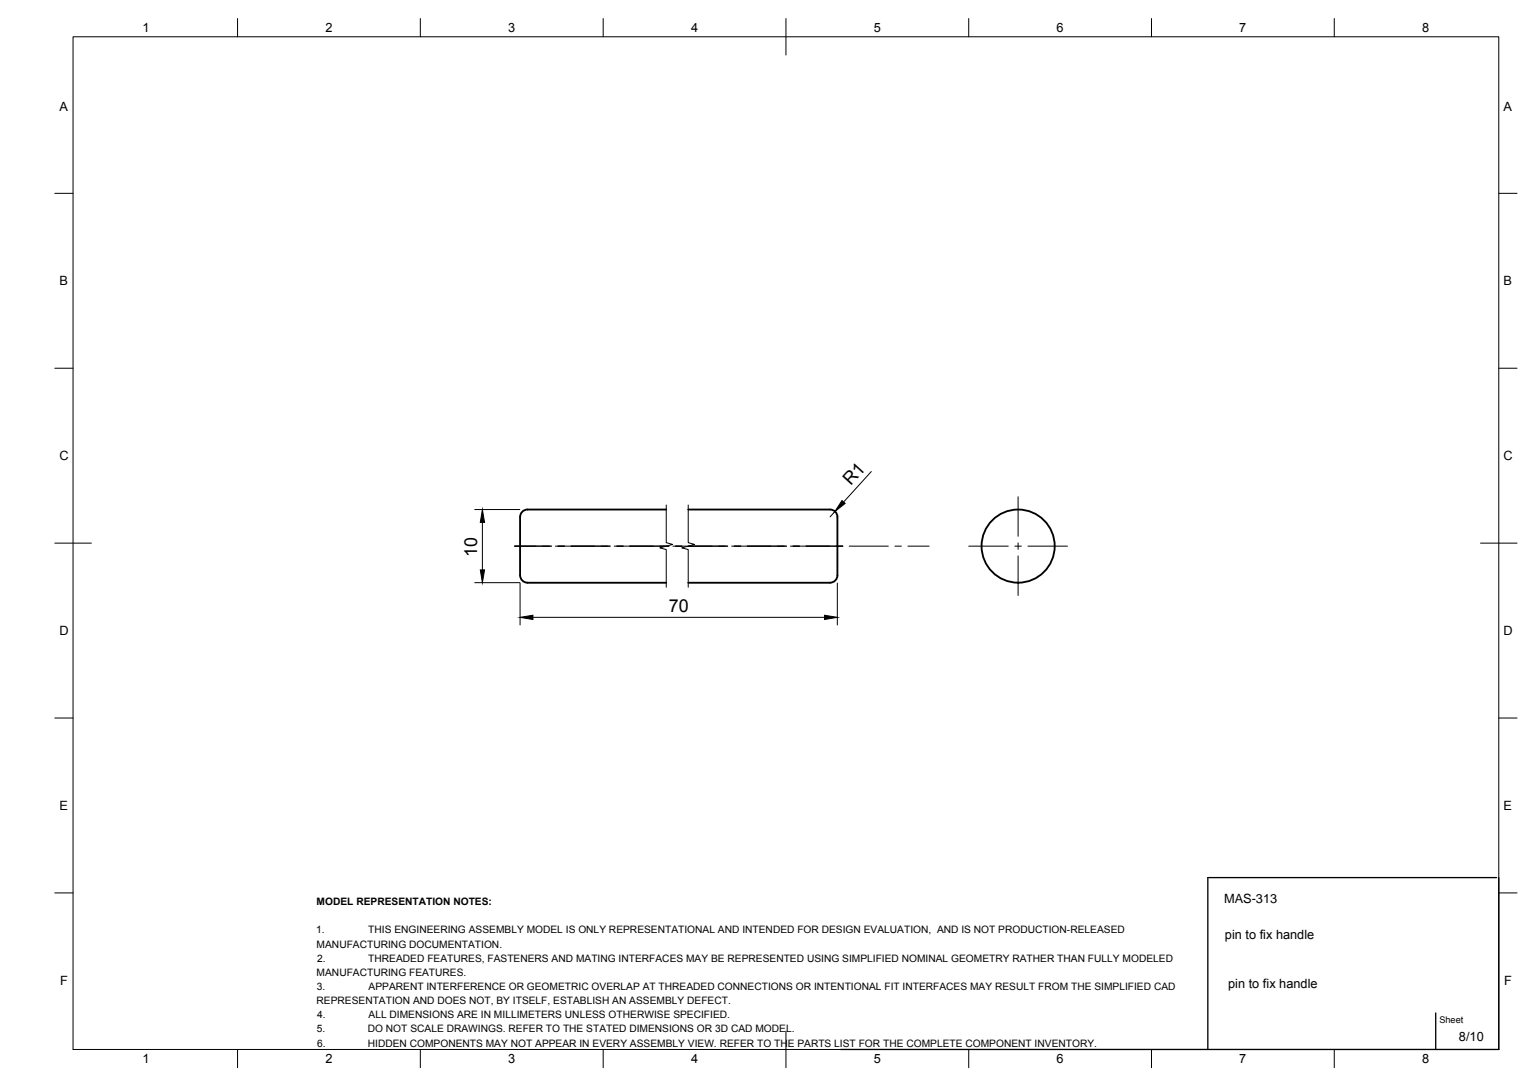
ISO-10303-21;
HEADER;
FILE_DESCRIPTION (('STEP AP214'),
    '1' );
FILE_NAME ('pin to fix handle.step',
    '2026-10-06T09:36:00',
    ( '' ),
    ( '' ),
    'SwSTEP 2.0',
    'SolidWorks 2025',
    '' );
FILE_SCHEMA (( 'AUTOMOTIVE_DESIGN' ));
ENDSEC;

DATA;
#87=VECTOR ( 'NONE', #10625, 1000.000000000000000 ) ;
#136=AXIS2_PLACEMENT_3D ( 'NONE', #2557, #579, #5269 ) ;
#167=DIRECTION ( 'NONE',  ( 1.000000000000000000, -1.876626137810916309E-30, 2.081668171172161734E-17 ) ) ;
#230=( LENGTH_UNIT ( ) NAMED_UNIT ( * ) SI_UNIT ( .MILLI., .METRE. ) );
#266=VECTOR ( 'NONE', #3751, 1000.000000000000000 ) ;
#291=PLANE ( 'NONE',  #9364 ) ;
#310=CARTESIAN_POINT ( 'NONE',  ( -823.8285638327238303, 78.67432280806536937, -89.68077099980398259 ) ) ;
#349=EDGE_CURVE ( 'NONE', #7831, #3787, #3152, .T. ) ;
#417=DIRECTION ( 'NONE',  ( 2.081668171172161734E-17, 4.930380657631307143E-31, -1.000000000000000000 ) ) ;
#440=CIRCLE ( 'NONE', #6189, 4.000000000000003553 ) ;
#493=EDGE_LOOP ( 'NONE', ( #7203, #9839, #8059, #6199 ) ) ;
#515=ORIENTED_EDGE ( 'NONE', *, *, #1701, .T. ) ;
#579=DIRECTION ( 'NONE',  ( -2.081668171172161734E-17, -4.930380657631307143E-31, 1.000000000000000000 ) ) ;
#638=CIRCLE ( 'NONE', #2031, 1.000000000000000888 ) ;
#710=DIRECTION ( 'NONE',  ( 1.000000000000000000, 0.000000000000000000, 0.000000000000000000 ) ) ;
#807=EDGE_CURVE ( 'NONE', #7831, #11221, #10092, .T. ) ;
#835=AXIS2_PLACEMENT_3D ( 'NONE', #1633, #2618, #6521 ) ;
#869=DIRECTION ( 'NONE',  ( 1.000000000000000000, -1.876626137810916309E-30, 2.081668171172161734E-17 ) ) ;
#886=ORIENTED_EDGE ( 'NONE', *, *, #1701, .F. ) ;
#924=LINE ( 'NONE', #5726, #266 ) ;
#977=DIRECTION ( 'NONE',  ( 1.000000000000000000, 0.000000000000000000, 0.000000000000000000 ) ) ;
#1010=CARTESIAN_POINT ( 'NONE',  ( -827.8285638327242850, 78.67432280806536937, -90.68077099980378364 ) ) ;
#1092=ORIENTED_EDGE ( 'NONE', *, *, #349, .F. ) ;
#1112=CARTESIAN_POINT ( 'NONE',  ( -818.8285638327247398, 78.67432280806536937, -158.6807709998041673 ) ) ;
#1184=SHAPE_REPRESENTATION_RELATIONSHIP ( 'NONE' , 'NONE' ,  #4872, #6043 ) ;
#1237=PRESENTATION_STYLE_ASSIGNMENT (( #7913 ) ) ;
#1300=DIRECTION ( 'NONE',  ( 1.000000000000000000, 0.000000000000000000, 0.000000000000000000 ) ) ;
#1388=ADVANCED_FACE ( 'NONE', ( #3889 ), #291, .F. ) ;
#1476=AXIS2_PLACEMENT_3D ( 'NONE', #10075, #7237, #11202 ) ;
#1505=ORIENTED_EDGE ( 'NONE', *, *, #349, .T. ) ;
#1609=CIRCLE ( 'NONE', #4593, 1.000000000000000888 ) ;
#1633=CARTESIAN_POINT ( 'NONE',  ( -823.8285638327242850, 78.67432280806536937, -90.68077099980378364 ) ) ;
#1659=CIRCLE ( 'NONE', #8766, 1.000000000000000888 ) ;
#1663=EDGE_LOOP ( 'NONE', ( #9512, #6396, #1868, #515 ) ) ;
#1669=CARTESIAN_POINT ( 'NONE',  ( -823.8285638327247398, 78.67432280806536937, -158.6807709998041673 ) ) ;
#1701=EDGE_CURVE ( 'NONE', #6923, #10076, #8157, .T. ) ;
#1727=ORIENTED_EDGE ( 'NONE', *, *, #11837, .F. ) ;
#1868=ORIENTED_EDGE ( 'NONE', *, *, #2750, .T. ) ;
#1872=PRODUCT_DEFINITION ( 'UNKNOWN', '', #5446, #1966 ) ;
#1966=PRODUCT_DEFINITION_CONTEXT ( 'detailed design', #7796, 'design' ) ;
#1972=AXIS2_PLACEMENT_3D ( 'NONE', #1669, #2530, #11129 ) ;
#2031=AXIS2_PLACEMENT_3D ( 'NONE', #6574, #2608, #7434 ) ;
#2069=EDGE_CURVE ( 'NONE', #10717, #3207, #440, .T. ) ;
#2234=CYLINDRICAL_SURFACE ( 'NONE', #9598, 5.000000000000115463 ) ;
#2273=CIRCLE ( 'NONE', #11162, 4.000000000000003553 ) ;
#2346=CARTESIAN_POINT ( 'NONE',  ( -823.8285638327245124, 78.67432280806536937, -159.6807709998044800 ) ) ;
#2363=( GEOMETRIC_REPRESENTATION_CONTEXT ( 3 ) GLOBAL_UNCERTAINTY_ASSIGNED_CONTEXT ( ( #10663 ) ) GLOBAL_UNIT_ASSIGNED_CONTEXT ( ( #230, #3198, #4081 ) ) REPRESENTATION_CONTEXT ( 'NONE', 'WORKASPACE' ) );
#2380=CARTESIAN_POINT ( 'NONE',  ( -818.8285638327237166, 78.67432280806536937, -89.68077099980398259 ) ) ;
#2394=FILL_AREA_STYLE ('',( #5928 ) ) ;
#2489=EDGE_LOOP ( 'NONE', ( #2863, #8978, #5125, #1092 ) ) ;
#2530=DIRECTION ( 'NONE',  ( -2.081668171172161734E-17, -4.930380657631307143E-31, 1.000000000000000000 ) ) ;
#2557=CARTESIAN_POINT ( 'NONE',  ( -823.8285638327247398, 78.67432280806536937, -158.6807709998041673 ) ) ;
#2608=DIRECTION ( 'NONE',  ( 1.224646799147376133E-16, 1.000000000000000000, 4.955873740258437191E-31 ) ) ;
#2618=DIRECTION ( 'NONE',  ( 2.081668171172161734E-17, 4.930380657631307143E-31, -1.000000000000000000 ) ) ;
#2750=EDGE_CURVE ( 'NONE', #11221, #6923, #924, .T. ) ;
#2778=DIRECTION ( 'NONE',  ( -2.081668171172161734E-17, -4.930380657631308019E-31, 1.000000000000000000 ) ) ;
#2790=CARTESIAN_POINT ( 'NONE',  ( -827.8285638327238303, 78.67432280806536937, -89.68077099980398259 ) ) ;
#2863=ORIENTED_EDGE ( 'NONE', *, *, #10666, .F. ) ;
#2903=EDGE_CURVE ( 'NONE', #11221, #8948, #1659, .T. ) ;
#3006=DIRECTION ( 'NONE',  ( 1.000000000000000000, -1.026341648675396322E-47, 2.081668171172161734E-17 ) ) ;
#3015=DIRECTION ( 'NONE',  ( 1.000000000000000000, 0.000000000000000000, 0.000000000000000000 ) ) ;
#3104=TOROIDAL_SURFACE ( 'NONE', #136, 4.000000000000045297, 1.000000000000000000 ) ;
#3152=CIRCLE ( 'NONE', #11256, 1.000000000000000888 ) ;
#3198=( NAMED_UNIT ( * ) PLANE_ANGLE_UNIT ( ) SI_UNIT ( $, .RADIAN. ) );
#3207=VERTEX_POINT ( 'NONE', #5427 ) ;
#3215=CARTESIAN_POINT ( 'NONE',  ( -823.8285638327242850, 78.67432280806536937, -90.68077099980378364 ) ) ;
#3400=ORIENTED_EDGE ( 'NONE', *, *, #2069, .T. ) ;
#3449=AXIS2_PLACEMENT_3D ( 'NONE', #7914, #9817, #5175 ) ;
#3543=DIRECTION ( 'NONE',  ( -2.081668171172161734E-17, -4.930380657631307143E-31, 1.000000000000000000 ) ) ;
#3642=FACE_OUTER_BOUND ( 'NONE', #1663, .T. ) ;
#3643=EDGE_LOOP ( 'NONE', ( #11417, #7051, #4704, #5616 ) ) ;
#3745=CARTESIAN_POINT ( 'NONE',  ( -823.8285638327247398, 78.67432280806536937, -158.6807709998041673 ) ) ;
#3751=DIRECTION ( 'NONE',  ( 2.081668171172161734E-17, 4.930380657631307143E-31, -1.000000000000000000 ) ) ;
#3787=VERTEX_POINT ( 'NONE', #7173 ) ;
#3807=ADVANCED_FACE ( 'NONE', ( #10268 ), #10840, .T. ) ;
#3889=FACE_OUTER_BOUND ( 'NONE', #4143, .T. ) ;
#3982=MANIFOLD_SOLID_BREP ( 'Fillet6', #4544 ) ;
#4081=( NAMED_UNIT ( * ) SI_UNIT ( $, .STERADIAN. ) SOLID_ANGLE_UNIT ( ) );
#4143=EDGE_LOOP ( 'NONE', ( #10187, #3400 ) ) ;
#4253=CARTESIAN_POINT ( 'NONE',  ( -823.8285638327238303, 78.67432280806536937, -89.68077099980398259 ) ) ;
#4432=DIRECTION ( 'NONE',  ( 1.000000000000000000, 0.000000000000000000, 0.000000000000000000 ) ) ;
#4501=AXIS2_PLACEMENT_3D ( 'NONE', #3215, #4892, #5819 ) ;
#4518=AXIS2_PLACEMENT_3D ( 'NONE', #11410, #6710, #3006 ) ;
#4544=CLOSED_SHELL ( 'NONE', ( #4609, #3807, #12155, #11684, #8450, #1388, #10453, #8041 ) ) ;
#4593=AXIS2_PLACEMENT_3D ( 'NONE', #10809, #8718, #7039 ) ;
#4609=ADVANCED_FACE ( 'NONE', ( #7576 ), #9837, .T. ) ;
#4626=CARTESIAN_POINT ( 'NONE',  ( -823.8285638327247398, 78.67432280806536937, -158.6807709998041673 ) ) ;
#4687=DIRECTION ( 'NONE',  ( 1.000000000000000000, 0.000000000000000000, 0.000000000000000000 ) ) ;
#4693=UNCERTAINTY_MEASURE_WITH_UNIT (LENGTH_MEASURE( 1.000000000000000082E-05 ), #8076, 'distance_accuracy_value', 'NONE');
#4699=CIRCLE ( 'NONE', #9621, 5.000000000000115463 ) ;
#4704=ORIENTED_EDGE ( 'NONE', *, *, #10020, .T. ) ;
#4754=FACE_OUTER_BOUND ( 'NONE', #8581, .T. ) ;
#4872=SHAPE_REPRESENTATION ( 'pin to fix handle', ( #11957 ), #10774 ) ;
#4885=EDGE_CURVE ( 'NONE', #3207, #10076, #1609, .T. ) ;
#4892=DIRECTION ( 'NONE',  ( -2.081668171172161734E-17, -4.930380657631307143E-31, 1.000000000000000000 ) ) ;
#5007=FACE_OUTER_BOUND ( 'NONE', #3643, .T. ) ;
#5035=AXIS2_PLACEMENT_3D ( 'NONE', #2346, #10626, #1300 ) ;
#5051=SURFACE_STYLE_FILL_AREA ( #2394 ) ;
#5118=STYLED_ITEM ( 'NONE', ( #1237 ), #3982 ) ;
#5125=ORIENTED_EDGE ( 'NONE', *, *, #11852, .F. ) ;
#5157=ORIENTED_EDGE ( 'NONE', *, *, #807, .F. ) ;
#5175=DIRECTION ( 'NONE',  ( 1.000000000000000000, 0.000000000000000000, 0.000000000000000000 ) ) ;
#5269=DIRECTION ( 'NONE',  ( 1.000000000000000000, -1.026341648675396322E-47, 2.081668171172161734E-17 ) ) ;
#5427=CARTESIAN_POINT ( 'NONE',  ( -819.8285638327245124, 78.67432280806536937, -159.6807709998044800 ) ) ;
#5446=PRODUCT_DEFINITION_FORMATION_WITH_SPECIFIED_SOURCE ( 'ANY', '', #7932, .NOT_KNOWN. ) ;
#5583=CARTESIAN_POINT ( 'NONE',  ( -818.8285638327242850, 78.67432280806536937, -90.68077099980378364 ) ) ;
#5590=DIRECTION ( 'NONE',  ( 2.081668171172161734E-17, 4.930380657631307143E-31, -1.000000000000000000 ) ) ;
#5616=ORIENTED_EDGE ( 'NONE', *, *, #2750, .F. ) ;
#5726=CARTESIAN_POINT ( 'NONE',  ( -828.8285638327239440, 78.67432280806536937, -89.68077099980398259 ) ) ;
#5735=PLANE ( 'NONE',  #7666 ) ;
#5784=ORIENTED_EDGE ( 'NONE', *, *, #11852, .T. ) ;
#5819=DIRECTION ( 'NONE',  ( 1.000000000000000000, -1.026341648675396322E-47, 2.081668171172161734E-17 ) ) ;
#5857=DIRECTION ( 'NONE',  ( -2.081668171172161734E-17, -4.930380657631308019E-31, 1.000000000000000000 ) ) ;
#5864=( NAMED_UNIT ( * ) PLANE_ANGLE_UNIT ( ) SI_UNIT ( $, .RADIAN. ) );
#5928=FILL_AREA_STYLE_COLOUR ( '', #9661 ) ;
#5979=EDGE_CURVE ( 'NONE', #10717, #6923, #638, .T. ) ;
#6032=CIRCLE ( 'NONE', #5035, 4.000000000000003553 ) ;
#6043=ADVANCED_BREP_SHAPE_REPRESENTATION ( '', ( #3982, #11957 ), #10774 ) ;
#6111=MECHANICAL_DESIGN_GEOMETRIC_PRESENTATION_REPRESENTATION('',(#5118),#2363);
#6132=APPLICATION_CONTEXT ( 'automotive_design' ) ;
#6189=AXIS2_PLACEMENT_3D ( 'NONE', #7587, #11482, #3015 ) ;
#6199=ORIENTED_EDGE ( 'NONE', *, *, #4885, .F. ) ;
#6267=CARTESIAN_POINT ( 'NONE',  ( -828.8285638327242850, 78.67432280806536937, -90.68077099980378364 ) ) ;
#6396=ORIENTED_EDGE ( 'NONE', *, *, #807, .T. ) ;
#6521=DIRECTION ( 'NONE',  ( 1.000000000000000000, 0.000000000000000000, 0.000000000000000000 ) ) ;
#6569=DIRECTION ( 'NONE',  ( 1.224646799147376133E-16, 1.000000000000000000, 4.955873740258437191E-31 ) ) ;
#6574=CARTESIAN_POINT ( 'NONE',  ( -827.8285638327247398, 78.67432280806536937, -158.6807709998041673 ) ) ;
#6624=ORIENTED_EDGE ( 'NONE', *, *, #2903, .F. ) ;
#6710=DIRECTION ( 'NONE',  ( -2.081668171172161734E-17, -4.930380657631307143E-31, 1.000000000000000000 ) ) ;
#6808=DIRECTION ( 'NONE',  ( -1.000000000000000000, 0.000000000000000000, 0.000000000000000000 ) ) ;
#6838=CARTESIAN_POINT ( 'NONE',  ( -819.8285638327242850, 78.67432280806536937, -90.68077099980378364 ) ) ;
#6866=TOROIDAL_SURFACE ( 'NONE', #4501, 4.000000000000045297, 1.000000000000000000 ) ;
#6889=EDGE_CURVE ( 'NONE', #7831, #10076, #11496, .T. ) ;
#6923=VERTEX_POINT ( 'NONE', #9178 ) ;
#7039=DIRECTION ( 'NONE',  ( 1.000000000000000000, 0.000000000000000000, 0.000000000000000000 ) ) ;
#7051=ORIENTED_EDGE ( 'NONE', *, *, #6889, .T. ) ;
#7173=CARTESIAN_POINT ( 'NONE',  ( -819.8285638327238303, 78.67432280806536937, -89.68077099980398259 ) ) ;
#7203=ORIENTED_EDGE ( 'NONE', *, *, #2069, .F. ) ;
#7237=DIRECTION ( 'NONE',  ( 2.081668171172161734E-17, 4.930380657631307143E-31, -1.000000000000000000 ) ) ;
#7380=EDGE_LOOP ( 'NONE', ( #8495, #1727, #7424, #886 ) ) ;
#7397=DIRECTION ( 'NONE',  ( -2.081668171172161734E-17, -4.930380657631307143E-31, 1.000000000000000000 ) ) ;
#7423=CYLINDRICAL_SURFACE ( 'NONE', #1476, 5.000000000000115463 ) ;
#7424=ORIENTED_EDGE ( 'NONE', *, *, #4885, .T. ) ;
#7434=DIRECTION ( 'NONE',  ( -1.000000000000000000, 0.000000000000000000, 0.000000000000000000 ) ) ;
#7439=DIRECTION ( 'NONE',  ( 1.000000000000000000, 0.000000000000000000, 0.000000000000000000 ) ) ;
#7576=FACE_OUTER_BOUND ( 'NONE', #2489, .T. ) ;
#7587=CARTESIAN_POINT ( 'NONE',  ( -823.8285638327245124, 78.67432280806536937, -159.6807709998044800 ) ) ;
#7637=SHAPE_DEFINITION_REPRESENTATION ( #8521, #4872 ) ;
#7658=EDGE_CURVE ( 'NONE', #8948, #3787, #2273, .T. ) ;
#7666=AXIS2_PLACEMENT_3D ( 'NONE', #11300, #2778, #869 ) ;
#7796=APPLICATION_CONTEXT ( 'automotive_design' ) ;
#7831=VERTEX_POINT ( 'NONE', #5583 ) ;
#7913=SURFACE_STYLE_USAGE ( .BOTH. , #10743 ) ;
#7914=CARTESIAN_POINT ( 'NONE',  ( -823.8285638327238303, 78.67432280806536937, -89.68077099980398259 ) ) ;
#7932=PRODUCT ( 'pin to fix handle', 'pin to fix handle', '', ( #11342 ) ) ;
#7955=DIRECTION ( 'NONE',  ( 1.000000000000000000, 0.000000000000000000, 0.000000000000000000 ) ) ;
#8041=ADVANCED_FACE ( 'NONE', ( #10822 ), #6866, .T. ) ;
#8059=ORIENTED_EDGE ( 'NONE', *, *, #10020, .F. ) ;
#8076=( LENGTH_UNIT ( ) NAMED_UNIT ( * ) SI_UNIT ( .MILLI., .METRE. ) );
#8157=CIRCLE ( 'NONE', #9541, 5.000000000000115463 ) ;
#8196=CARTESIAN_POINT ( 'NONE',  ( -827.8285638327245124, 78.67432280806536937, -159.6807709998044800 ) ) ;
#8323=FACE_OUTER_BOUND ( 'NONE', #7380, .T. ) ;
#8450=ADVANCED_FACE ( 'NONE', ( #4754 ), #5735, .T. ) ;
#8495=ORIENTED_EDGE ( 'NONE', *, *, #5979, .F. ) ;
#8498=DIRECTION ( 'NONE',  ( -1.000000000000000000, 0.000000000000000000, 0.000000000000000000 ) ) ;
#8521=PRODUCT_DEFINITION_SHAPE ( 'NONE', 'NONE',  #1872 ) ;
#8581=EDGE_LOOP ( 'NONE', ( #5784, #11546 ) ) ;
#8718=DIRECTION ( 'NONE',  ( -1.876626137810916309E-30, -1.000000000000000000, -4.930380657631307143E-31 ) ) ;
#8766=AXIS2_PLACEMENT_3D ( 'NONE', #1010, #6569, #8498 ) ;
#8948=VERTEX_POINT ( 'NONE', #2790 ) ;
#8978=ORIENTED_EDGE ( 'NONE', *, *, #2903, .T. ) ;
#9048=CARTESIAN_POINT ( 'NONE',  ( 0.000000000000000000, 0.000000000000000000, 0.000000000000000000 ) ) ;
#9105=CARTESIAN_POINT ( 'NONE',  ( -823.8285638327242850, 78.67432280806536937, -90.68077099980378364 ) ) ;
#9178=CARTESIAN_POINT ( 'NONE',  ( -828.8285638327247398, 78.67432280806536937, -158.6807709998041673 ) ) ;
#9364=AXIS2_PLACEMENT_3D ( 'NONE', #9577, #5857, #167 ) ;
#9440=DIRECTION ( 'NONE',  ( -1.876626137810916309E-30, -1.000000000000000000, -4.930380657631307143E-31 ) ) ;
#9512=ORIENTED_EDGE ( 'NONE', *, *, #6889, .F. ) ;
#9541=AXIS2_PLACEMENT_3D ( 'NONE', #4626, #3543, #4432 ) ;
#9577=CARTESIAN_POINT ( 'NONE',  ( -823.8285638327245124, 78.67432280806536937, -159.6807709998044800 ) ) ;
#9598=AXIS2_PLACEMENT_3D ( 'NONE', #310, #417, #6808 ) ;
#9621=AXIS2_PLACEMENT_3D ( 'NONE', #9105, #5590, #710 ) ;
#9661=COLOUR_RGB ( '', 0.72549020, 0.75294118, 0.79215686) ;
#9817=DIRECTION ( 'NONE',  ( -2.081668171172161734E-17, -4.930380657631307143E-31, 1.000000000000000000 ) ) ;
#9837=TOROIDAL_SURFACE ( 'NONE', #4518, 4.000000000000045297, 1.000000000000000000 ) ;
#9839=ORIENTED_EDGE ( 'NONE', *, *, #5979, .T. ) ;
#9973=CIRCLE ( 'NONE', #3449, 4.000000000000003553 ) ;
#10001=EDGE_LOOP ( 'NONE', ( #6624, #5157, #1505, #11857 ) ) ;
#10020=EDGE_CURVE ( 'NONE', #10076, #6923, #11591, .T. ) ;
#10075=CARTESIAN_POINT ( 'NONE',  ( -823.8285638327238303, 78.67432280806536937, -89.68077099980398259 ) ) ;
#10076=VERTEX_POINT ( 'NONE', #1112 ) ;
#10092=CIRCLE ( 'NONE', #835, 5.000000000000115463 ) ;
#10187=ORIENTED_EDGE ( 'NONE', *, *, #11837, .T. ) ;
#10268=FACE_OUTER_BOUND ( 'NONE', #493, .T. ) ;
#10453=ADVANCED_FACE ( 'NONE', ( #8323 ), #3104, .T. ) ;
#10625=DIRECTION ( 'NONE',  ( 2.081668171172161734E-17, 4.930380657631307143E-31, -1.000000000000000000 ) ) ;
#10626=DIRECTION ( 'NONE',  ( 2.081668171172161734E-17, 4.930380657631307143E-31, -1.000000000000000000 ) ) ;
#10627=( NAMED_UNIT ( * ) SI_UNIT ( $, .STERADIAN. ) SOLID_ANGLE_UNIT ( ) );
#10663=UNCERTAINTY_MEASURE_WITH_UNIT (LENGTH_MEASURE( 1.000000000000000082E-05 ), #230, 'distance_accuracy_value', 'NONE');
#10666=EDGE_CURVE ( 'NONE', #11221, #7831, #4699, .T. ) ;
#10717=VERTEX_POINT ( 'NONE', #8196 ) ;
#10743=SURFACE_SIDE_STYLE ('',( #5051 ) ) ;
#10774=( GEOMETRIC_REPRESENTATION_CONTEXT ( 3 ) GLOBAL_UNCERTAINTY_ASSIGNED_CONTEXT ( ( #4693 ) ) GLOBAL_UNIT_ASSIGNED_CONTEXT ( ( #8076, #5864, #10627 ) ) REPRESENTATION_CONTEXT ( 'NONE', 'WORKASPACE' ) );
#10809=CARTESIAN_POINT ( 'NONE',  ( -819.8285638327247398, 78.67432280806536937, -158.6807709998041673 ) ) ;
#10822=FACE_OUTER_BOUND ( 'NONE', #10001, .T. ) ;
#10840=TOROIDAL_SURFACE ( 'NONE', #1972, 4.000000000000045297, 1.000000000000000000 ) ;
#10904=DIRECTION ( 'NONE',  ( 0.000000000000000000, 0.000000000000000000, 1.000000000000000000 ) ) ;
#11129=DIRECTION ( 'NONE',  ( 1.000000000000000000, -1.026341648675396322E-47, 2.081668171172161734E-17 ) ) ;
#11162=AXIS2_PLACEMENT_3D ( 'NONE', #4253, #12152, #7439 ) ;
#11202=DIRECTION ( 'NONE',  ( -1.000000000000000000, 0.000000000000000000, 0.000000000000000000 ) ) ;
#11221=VERTEX_POINT ( 'NONE', #6267 ) ;
#11256=AXIS2_PLACEMENT_3D ( 'NONE', #6838, #9440, #977 ) ;
#11300=CARTESIAN_POINT ( 'NONE',  ( -823.8285638327238303, 78.67432280806536937, -89.68077099980398259 ) ) ;
#11342=PRODUCT_CONTEXT ( 'NONE', #6132, 'mechanical' ) ;
#11410=CARTESIAN_POINT ( 'NONE',  ( -823.8285638327242850, 78.67432280806536937, -90.68077099980378364 ) ) ;
#11417=ORIENTED_EDGE ( 'NONE', *, *, #10666, .T. ) ;
#11482=DIRECTION ( 'NONE',  ( 2.081668171172161734E-17, 4.930380657631307143E-31, -1.000000000000000000 ) ) ;
#11496=LINE ( 'NONE', #2380, #87 ) ;
#11546=ORIENTED_EDGE ( 'NONE', *, *, #7658, .T. ) ;
#11591=CIRCLE ( 'NONE', #11978, 5.000000000000115463 ) ;
#11684=ADVANCED_FACE ( 'NONE', ( #3642 ), #7423, .T. ) ;
#11837=EDGE_CURVE ( 'NONE', #3207, #10717, #6032, .T. ) ;
#11852=EDGE_CURVE ( 'NONE', #3787, #8948, #9973, .T. ) ;
#11857=ORIENTED_EDGE ( 'NONE', *, *, #7658, .F. ) ;
#11957=AXIS2_PLACEMENT_3D ( 'NONE', #9048, #10904, #7955 ) ;
#11978=AXIS2_PLACEMENT_3D ( 'NONE', #3745, #7397, #4687 ) ;
#12152=DIRECTION ( 'NONE',  ( -2.081668171172161734E-17, -4.930380657631307143E-31, 1.000000000000000000 ) ) ;
#12155=ADVANCED_FACE ( 'NONE', ( #5007 ), #2234, .T. ) ;
ENDSEC;
END-ISO-10303-21;
